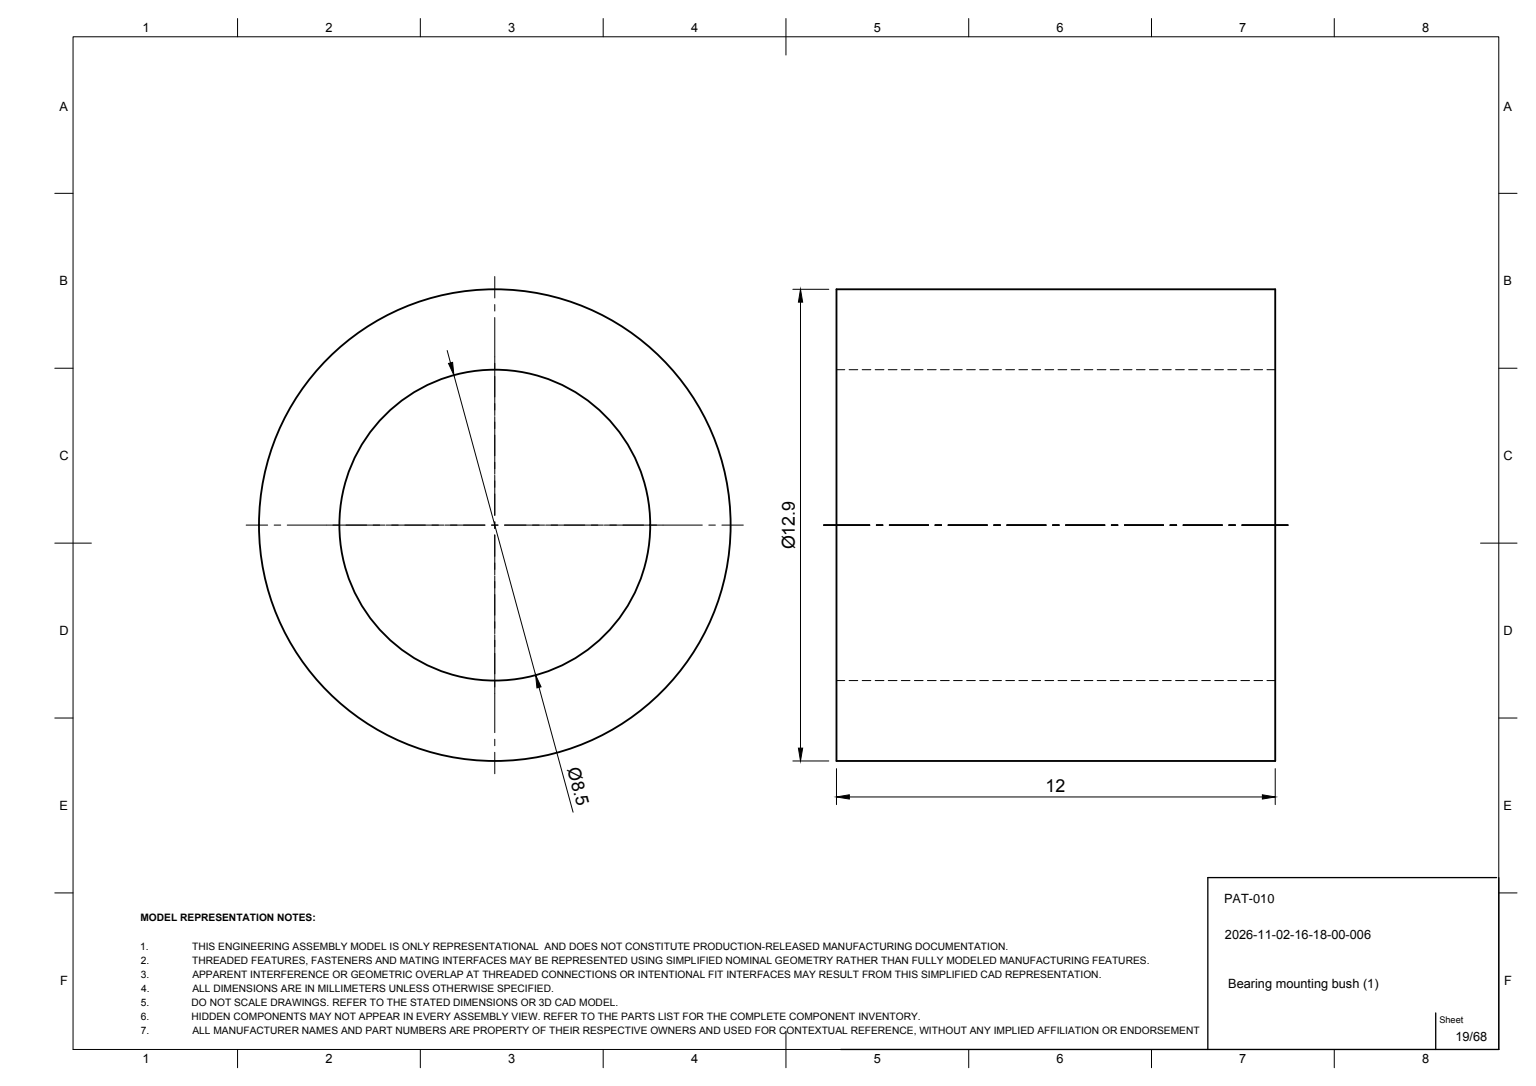
ISO-10303-21;
HEADER;
/* Generated by software containing ST-Developer
 * from STEP Tools, Inc. (www.steptools.com) 
 */

FILE_DESCRIPTION(
/* description */ ('Belt conveyor head drive unit'),
/* implementation_level */ '2;1');

FILE_NAME(
/* name */ 'Bearing mounting bush (1).step',
/* time_stamp */ '2026-10-28T03:26:19-07:00',
/* author */ (''),
/* organization */ (''),
/* preprocessor_version */ 'ST-DEVELOPER v20.2',
/* originating_system */ 'Autodesk Translation Framework v15.17.0.0',
/* authorisation */ '');

FILE_SCHEMA (('AUTOMOTIVE_DESIGN { 1 0 10303 214 3 1 1 }'));
ENDSEC;

DATA;
#10=MECHANICAL_DESIGN_GEOMETRIC_PRESENTATION_REPRESENTATION('',(#865),#27069);
#727=SHAPE_REPRESENTATION_RELATIONSHIP('SRR','None',#27371,#796);
#796=ADVANCED_BREP_SHAPE_REPRESENTATION('',(#950),#27013);
#865=STYLED_ITEM('',(#27797),#950);
#950=MANIFOLD_SOLID_BREP('Body1',#13730);
#1109=FACE_BOUND('',#2757,.T.);
#1110=FACE_BOUND('',#2759,.T.);
#1387=PLANE('',#15053);
#1388=PLANE('',#15054);
#1857=FACE_OUTER_BOUND('',#2754,.T.);
#1858=FACE_OUTER_BOUND('',#2755,.T.);
#1859=FACE_OUTER_BOUND('',#2756,.T.);
#1860=FACE_OUTER_BOUND('',#2758,.T.);
#2754=EDGE_LOOP('',(#9960,#9961,#9962,#9963));
#2755=EDGE_LOOP('',(#9964,#9965,#9966,#9967));
#2756=EDGE_LOOP('',(#9968));
#2757=EDGE_LOOP('',(#9969));
#2758=EDGE_LOOP('',(#9970));
#2759=EDGE_LOOP('',(#9971));
#3759=LINE('',#22054,#4551);
#3760=LINE('',#22060,#4552);
#4551=VECTOR('',#17669,0.425000000000001);
#4552=VECTOR('',#17676,0.645);
#5322=CIRCLE('',#15048,0.425000000000001);
#5323=CIRCLE('',#15049,0.425000000000001);
#5324=CIRCLE('',#15051,0.645);
#5325=CIRCLE('',#15052,0.645);
#6287=VERTEX_POINT('',#22051);
#6288=VERTEX_POINT('',#22053);
#6289=VERTEX_POINT('',#22057);
#6290=VERTEX_POINT('',#22059);
#7672=EDGE_CURVE('',#6287,#6287,#5322,.T.);
#7673=EDGE_CURVE('',#6287,#6288,#3759,.T.);
#7674=EDGE_CURVE('',#6288,#6288,#5323,.T.);
#7675=EDGE_CURVE('',#6289,#6289,#5324,.T.);
#7676=EDGE_CURVE('',#6289,#6290,#3760,.T.);
#7677=EDGE_CURVE('',#6290,#6290,#5325,.T.);
#9960=ORIENTED_EDGE('',*,*,#7672,.F.);
#9961=ORIENTED_EDGE('',*,*,#7673,.T.);
#9962=ORIENTED_EDGE('',*,*,#7674,.T.);
#9963=ORIENTED_EDGE('',*,*,#7673,.F.);
#9964=ORIENTED_EDGE('',*,*,#7675,.F.);
#9965=ORIENTED_EDGE('',*,*,#7676,.T.);
#9966=ORIENTED_EDGE('',*,*,#7677,.T.);
#9967=ORIENTED_EDGE('',*,*,#7676,.F.);
#9968=ORIENTED_EDGE('',*,*,#7675,.T.);
#9969=ORIENTED_EDGE('',*,*,#7672,.T.);
#9970=ORIENTED_EDGE('',*,*,#7677,.F.);
#9971=ORIENTED_EDGE('',*,*,#7674,.F.);
#12646=CYLINDRICAL_SURFACE('',#15047,0.425000000000001);
#12647=CYLINDRICAL_SURFACE('',#15050,0.645);
#13136=ADVANCED_FACE('',(#1857),#12646,.F.);
#13137=ADVANCED_FACE('',(#1858),#12647,.T.);
#13138=ADVANCED_FACE('',(#1859,#1109),#1387,.T.);
#13139=ADVANCED_FACE('',(#1860,#1110),#1388,.F.);
#13730=CLOSED_SHELL('',(#13136,#13137,#13138,#13139));
#15046=AXIS2_PLACEMENT_3D('',#22049,#17663,#17664);
#15047=AXIS2_PLACEMENT_3D('',#22050,#17665,#17666);
#15048=AXIS2_PLACEMENT_3D('',#22052,#17667,#17668);
#15049=AXIS2_PLACEMENT_3D('',#22055,#17670,#17671);
#15050=AXIS2_PLACEMENT_3D('',#22056,#17672,#17673);
#15051=AXIS2_PLACEMENT_3D('',#22058,#17674,#17675);
#15052=AXIS2_PLACEMENT_3D('',#22061,#17677,#17678);
#15053=AXIS2_PLACEMENT_3D('',#22062,#17679,#17680);
#15054=AXIS2_PLACEMENT_3D('',#22063,#17681,#17682);
#17663=DIRECTION('axis',(0.,0.,1.));
#17664=DIRECTION('refdir',(1.,0.,0.));
#17665=DIRECTION('center_axis',(0.,0.,1.));
#17666=DIRECTION('ref_axis',(1.,0.,0.));
#17667=DIRECTION('center_axis',(0.,0.,-1.));
#17668=DIRECTION('ref_axis',(1.,0.,0.));
#17669=DIRECTION('',(0.,0.,-1.));
#17670=DIRECTION('center_axis',(0.,0.,-1.));
#17671=DIRECTION('ref_axis',(1.,0.,0.));
#17672=DIRECTION('center_axis',(0.,0.,1.));
#17673=DIRECTION('ref_axis',(1.,0.,0.));
#17674=DIRECTION('center_axis',(0.,0.,1.));
#17675=DIRECTION('ref_axis',(1.,0.,0.));
#17676=DIRECTION('',(0.,0.,-1.));
#17677=DIRECTION('center_axis',(0.,0.,1.));
#17678=DIRECTION('ref_axis',(1.,0.,0.));
#17679=DIRECTION('center_axis',(0.,0.,1.));
#17680=DIRECTION('ref_axis',(1.,0.,0.));
#17681=DIRECTION('center_axis',(0.,0.,1.));
#17682=DIRECTION('ref_axis',(1.,0.,0.));
#22049=CARTESIAN_POINT('',(0.,0.,0.));
#22050=CARTESIAN_POINT('Origin',(11.7209100301812,4.,3.67));
#22051=CARTESIAN_POINT('',(11.2959100301812,4.,4.87));
#22052=CARTESIAN_POINT('Origin',(11.7209100301812,4.,4.87));
#22053=CARTESIAN_POINT('',(11.2959100301812,4.,3.67));
#22054=CARTESIAN_POINT('',(11.2959100301812,4.,3.67));
#22055=CARTESIAN_POINT('Origin',(11.7209100301812,4.,3.67));
#22056=CARTESIAN_POINT('Origin',(11.7209100301812,4.,3.67));
#22057=CARTESIAN_POINT('',(11.0759100301812,4.,4.87));
#22058=CARTESIAN_POINT('Origin',(11.7209100301812,4.,4.87));
#22059=CARTESIAN_POINT('',(11.0759100301812,4.,3.67));
#22060=CARTESIAN_POINT('',(11.0759100301812,4.,3.67));
#22061=CARTESIAN_POINT('Origin',(11.7209100301812,4.,3.67));
#22062=CARTESIAN_POINT('Origin',(11.7209100301812,4.,4.87));
#22063=CARTESIAN_POINT('Origin',(11.7209100301812,4.,3.67));
#26936=UNCERTAINTY_MEASURE_WITH_UNIT(LENGTH_MEASURE(0.001),#27070,
'DISTANCE_ACCURACY_VALUE',
'Maximum model space distance between geometric entities at asserted c
onnectivities');
#26992=UNCERTAINTY_MEASURE_WITH_UNIT(LENGTH_MEASURE(0.001),#27070,
'DISTANCE_ACCURACY_VALUE',
'Maximum model space distance between geometric entities at asserted c
onnectivities');
#27013=(
GEOMETRIC_REPRESENTATION_CONTEXT(3)
GLOBAL_UNCERTAINTY_ASSIGNED_CONTEXT((#26936))
GLOBAL_UNIT_ASSIGNED_CONTEXT((#27070,#27072,#27073))
REPRESENTATION_CONTEXT('','3D')
);
#27069=(
GEOMETRIC_REPRESENTATION_CONTEXT(3)
GLOBAL_UNCERTAINTY_ASSIGNED_CONTEXT((#26992))
GLOBAL_UNIT_ASSIGNED_CONTEXT((#27070,#27072,#27073))
REPRESENTATION_CONTEXT('','3D')
);
#27070=(
LENGTH_UNIT()
NAMED_UNIT(*)
SI_UNIT(.CENTI.,.METRE.)
);
#27072=(
NAMED_UNIT(*)
PLANE_ANGLE_UNIT()
SI_UNIT($,.RADIAN.)
);
#27073=(
NAMED_UNIT(*)
SI_UNIT($,.STERADIAN.)
SOLID_ANGLE_UNIT()
);
#27094=SHAPE_DEFINITION_REPRESENTATION(#27170,#27371);
#27170=PRODUCT_DEFINITION_SHAPE('',$,#27448);
#27371=SHAPE_REPRESENTATION('',(#15046),#27013);
#27427=PRODUCT_DEFINITION_CONTEXT('part definition',#27657,'design');
#27448=PRODUCT_DEFINITION('Bearing mounting bush (1)',
'Bearing mounting bush (1)',#27524,#27427);
#27524=PRODUCT_DEFINITION_FORMATION('',$,#27679);
#27657=APPLICATION_CONTEXT(
'Core Data for Automotive Mechanical Design Process');
#27658=PRODUCT_CONTEXT('part definition',#27657,'mechanical');
#27679=PRODUCT('Bearing mounting bush (1)','Bearing mounting bush (1)',
'Bearing mounting bush (1)',(#27658));
#27791=COLOUR_RGB('Grey',0.48,0.52,0.57);
#27792=FILL_AREA_STYLE_COLOUR('',#27791);
#27793=FILL_AREA_STYLE('',(#27792));
#27794=SURFACE_STYLE_FILL_AREA(#27793);
#27795=SURFACE_SIDE_STYLE('',(#27794));
#27796=SURFACE_STYLE_USAGE(.BOTH.,#27795);
#27797=PRESENTATION_STYLE_ASSIGNMENT((#27796));
ENDSEC;
END-ISO-10303-21;
